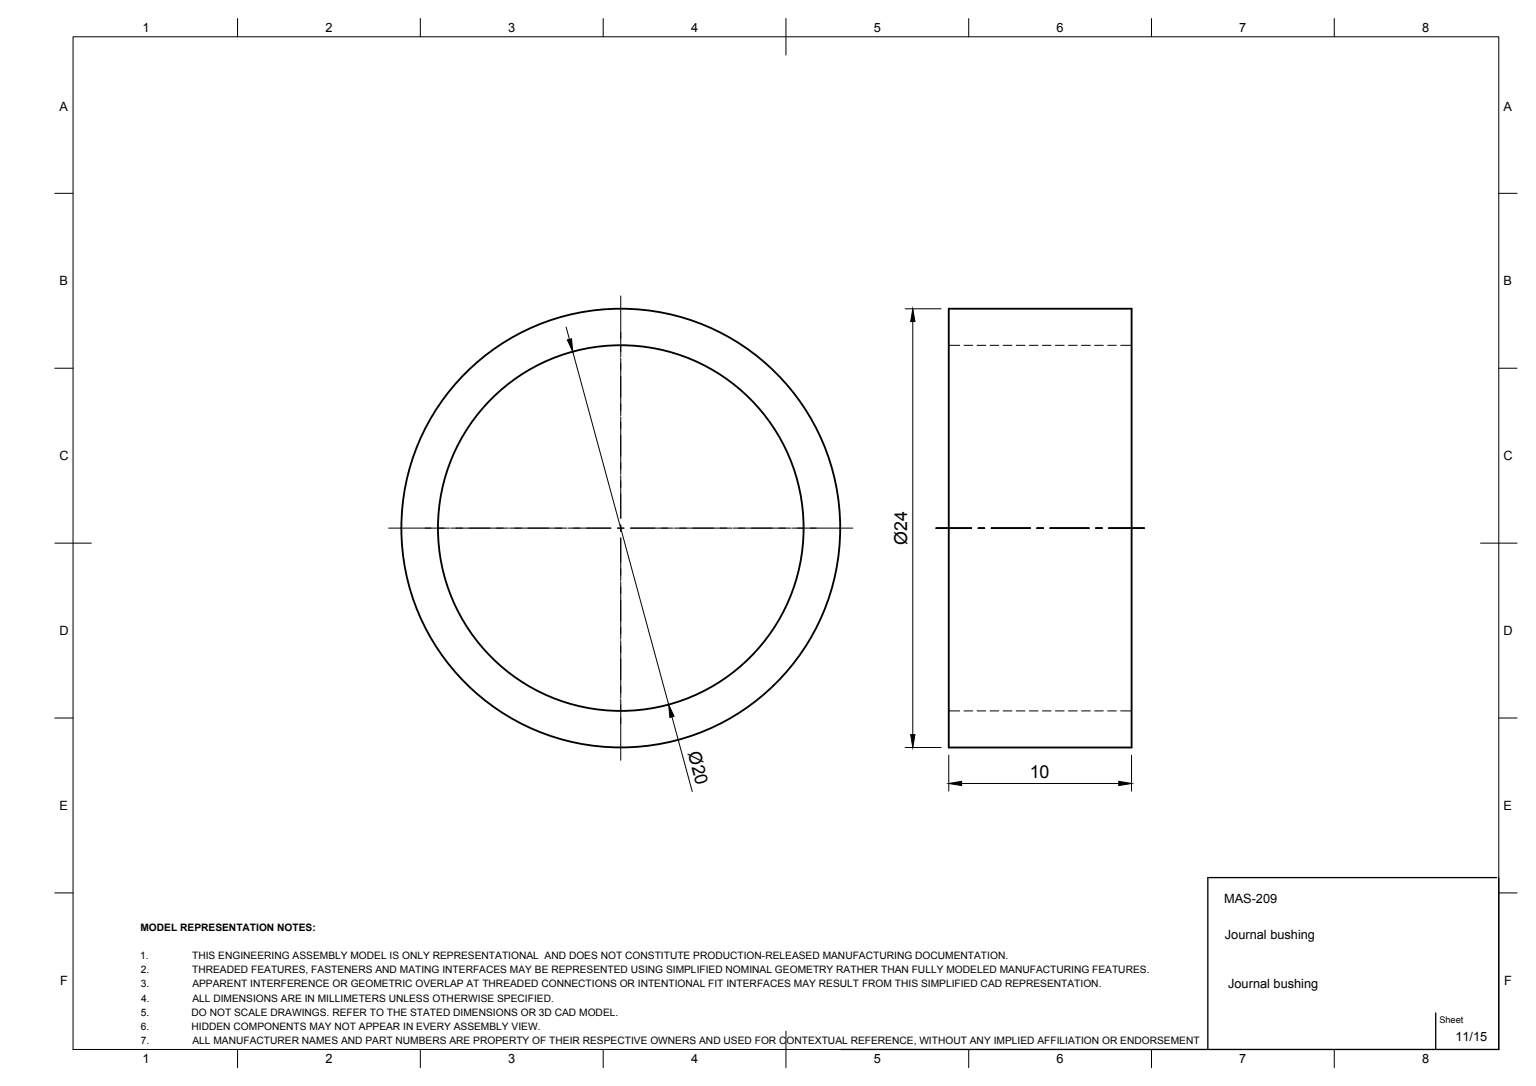
ISO-10303-21;
HEADER;
/* Generated by software containing ST-Developer
 * from STEP Tools, Inc. (www.steptools.com) 
 */

FILE_DESCRIPTION(
/* description */ ('Independent bearing-supported roller-ramp one-way clutch. Six logarit
hmic ramps with plain solid rollers, sprung guided plungers, native Co
il variants, removable shared keepers, rounded parallel key, shaft wit
h complete retaining lips, bronze journal/thrust support and bolted co
vers. Native rotor, roller planar/spin and plunger joints permit manua
l geometric engaged/released inspection. Automatic frictional torque s
witching/contact dynamics are not simulated; no capacity, hardness, fi
t, lubrication, speed, force or life rating. External input driver/cou
pling/anchors outside assembly.'),
/* implementation_level */ '2;1');

FILE_NAME(
/* name */ 'Journal bushing.step',
/* time_stamp */ '2026-11-08T07:04:38-08:00',
/* author */ (''),
/* organization */ (''),
/* preprocessor_version */ 'ST-DEVELOPER v20.2',
/* originating_system */ 'Autodesk Translation Framework v15.17.0.0',
/* authorisation */ '');

FILE_SCHEMA (('AUTOMOTIVE_DESIGN { 1 0 10303 214 3 1 1 }'));
ENDSEC;

DATA;
#10=MECHANICAL_DESIGN_GEOMETRIC_PRESENTATION_REPRESENTATION('',(#308),#99526);
#276=SHAPE_REPRESENTATION_RELATIONSHIP('SRR','None',#99633,#292);
#292=ADVANCED_BREP_SHAPE_REPRESENTATION('',(#324),#99518);
#308=STYLED_ITEM('',(#99720),#324);
#324=MANIFOLD_SOLID_BREP('Body1',#18278);
#430=FACE_BOUND('',#2664,.T.);
#431=FACE_BOUND('',#2666,.T.);
#579=PLANE('',#19601);
#580=PLANE('',#19602);
#1566=FACE_OUTER_BOUND('',#2661,.T.);
#1567=FACE_OUTER_BOUND('',#2662,.T.);
#1568=FACE_OUTER_BOUND('',#2663,.T.);
#1569=FACE_OUTER_BOUND('',#2665,.T.);
#2661=EDGE_LOOP('',(#16020,#16021,#16022,#16023));
#2662=EDGE_LOOP('',(#16024,#16025,#16026,#16027));
#2663=EDGE_LOOP('',(#16028));
#2664=EDGE_LOOP('',(#16029));
#2665=EDGE_LOOP('',(#16030));
#2666=EDGE_LOOP('',(#16031));
#3076=CIRCLE('',#19596,10.);
#3077=CIRCLE('',#19597,10.);
#3078=CIRCLE('',#19599,12.);
#3079=CIRCLE('',#19600,12.);
#5430=LINE('',#94854,#6334);
#5431=LINE('',#94860,#6335);
#6334=VECTOR('',#22867,10.);
#6335=VECTOR('',#22874,12.);
#8091=VERTEX_POINT('',#94851);
#8092=VERTEX_POINT('',#94853);
#8093=VERTEX_POINT('',#94857);
#8094=VERTEX_POINT('',#94859);
#10762=EDGE_CURVE('',#8091,#8091,#3076,.T.);
#10763=EDGE_CURVE('',#8091,#8092,#5430,.T.);
#10764=EDGE_CURVE('',#8092,#8092,#3077,.T.);
#10765=EDGE_CURVE('',#8093,#8093,#3078,.T.);
#10766=EDGE_CURVE('',#8093,#8094,#5431,.T.);
#10767=EDGE_CURVE('',#8094,#8094,#3079,.T.);
#16020=ORIENTED_EDGE('',*,*,#10762,.F.);
#16021=ORIENTED_EDGE('',*,*,#10763,.T.);
#16022=ORIENTED_EDGE('',*,*,#10764,.T.);
#16023=ORIENTED_EDGE('',*,*,#10763,.F.);
#16024=ORIENTED_EDGE('',*,*,#10765,.F.);
#16025=ORIENTED_EDGE('',*,*,#10766,.T.);
#16026=ORIENTED_EDGE('',*,*,#10767,.T.);
#16027=ORIENTED_EDGE('',*,*,#10766,.F.);
#16028=ORIENTED_EDGE('',*,*,#10765,.T.);
#16029=ORIENTED_EDGE('',*,*,#10762,.T.);
#16030=ORIENTED_EDGE('',*,*,#10767,.F.);
#16031=ORIENTED_EDGE('',*,*,#10764,.F.);
#17210=CYLINDRICAL_SURFACE('',#19595,10.);
#17211=CYLINDRICAL_SURFACE('',#19598,12.);
#18164=ADVANCED_FACE('',(#1566),#17210,.F.);
#18165=ADVANCED_FACE('',(#1567),#17211,.T.);
#18166=ADVANCED_FACE('',(#1568,#430),#579,.T.);
#18167=ADVANCED_FACE('',(#1569,#431),#580,.F.);
#18278=CLOSED_SHELL('',(#18164,#18165,#18166,#18167));
#19594=AXIS2_PLACEMENT_3D('',#94849,#22861,#22862);
#19595=AXIS2_PLACEMENT_3D('',#94850,#22863,#22864);
#19596=AXIS2_PLACEMENT_3D('',#94852,#22865,#22866);
#19597=AXIS2_PLACEMENT_3D('',#94855,#22868,#22869);
#19598=AXIS2_PLACEMENT_3D('',#94856,#22870,#22871);
#19599=AXIS2_PLACEMENT_3D('',#94858,#22872,#22873);
#19600=AXIS2_PLACEMENT_3D('',#94861,#22875,#22876);
#19601=AXIS2_PLACEMENT_3D('',#94862,#22877,#22878);
#19602=AXIS2_PLACEMENT_3D('',#94863,#22879,#22880);
#22861=DIRECTION('axis',(0.,0.,1.));
#22862=DIRECTION('refdir',(1.,0.,0.));
#22863=DIRECTION('center_axis',(0.,0.,1.));
#22864=DIRECTION('ref_axis',(1.,0.,0.));
#22865=DIRECTION('center_axis',(0.,0.,-1.));
#22866=DIRECTION('ref_axis',(1.,0.,0.));
#22867=DIRECTION('',(0.,0.,-1.));
#22868=DIRECTION('center_axis',(0.,0.,-1.));
#22869=DIRECTION('ref_axis',(1.,0.,0.));
#22870=DIRECTION('center_axis',(0.,0.,1.));
#22871=DIRECTION('ref_axis',(1.,0.,0.));
#22872=DIRECTION('center_axis',(0.,0.,1.));
#22873=DIRECTION('ref_axis',(1.,0.,0.));
#22874=DIRECTION('',(0.,0.,-1.));
#22875=DIRECTION('center_axis',(0.,0.,1.));
#22876=DIRECTION('ref_axis',(1.,0.,0.));
#22877=DIRECTION('center_axis',(0.,0.,1.));
#22878=DIRECTION('ref_axis',(1.,0.,0.));
#22879=DIRECTION('center_axis',(0.,0.,1.));
#22880=DIRECTION('ref_axis',(1.,0.,0.));
#94849=CARTESIAN_POINT('',(0.,0.,0.));
#94850=CARTESIAN_POINT('Origin',(0.,0.,0.));
#94851=CARTESIAN_POINT('',(-10.,-1.22464679914735E-15,10.));
#94852=CARTESIAN_POINT('Origin',(0.,0.,10.));
#94853=CARTESIAN_POINT('',(-10.,-1.22464679914735E-15,0.));
#94854=CARTESIAN_POINT('',(-10.,-1.22464679914735E-15,0.));
#94855=CARTESIAN_POINT('Origin',(0.,0.,0.));
#94856=CARTESIAN_POINT('Origin',(0.,0.,0.));
#94857=CARTESIAN_POINT('',(-12.,-1.46957615897682E-15,10.));
#94858=CARTESIAN_POINT('Origin',(0.,0.,10.));
#94859=CARTESIAN_POINT('',(-12.,-1.46957615897682E-15,0.));
#94860=CARTESIAN_POINT('',(-12.,-1.46957615897682E-15,0.));
#94861=CARTESIAN_POINT('Origin',(0.,0.,0.));
#94862=CARTESIAN_POINT('Origin',(0.,0.,10.));
#94863=CARTESIAN_POINT('Origin',(0.,0.,0.));
#99500=UNCERTAINTY_MEASURE_WITH_UNIT(LENGTH_MEASURE(0.01),#99527,
'DISTANCE_ACCURACY_VALUE',
'Maximum model space distance between geometric entities at asserted c
onnectivities');
#99508=UNCERTAINTY_MEASURE_WITH_UNIT(LENGTH_MEASURE(0.01),#99527,
'DISTANCE_ACCURACY_VALUE',
'Maximum model space distance between geometric entities at asserted c
onnectivities');
#99518=(
GEOMETRIC_REPRESENTATION_CONTEXT(3)
GLOBAL_UNCERTAINTY_ASSIGNED_CONTEXT((#99500))
GLOBAL_UNIT_ASSIGNED_CONTEXT((#99527,#99529,#99530))
REPRESENTATION_CONTEXT('','3D')
);
#99526=(
GEOMETRIC_REPRESENTATION_CONTEXT(3)
GLOBAL_UNCERTAINTY_ASSIGNED_CONTEXT((#99508))
GLOBAL_UNIT_ASSIGNED_CONTEXT((#99527,#99529,#99530))
REPRESENTATION_CONTEXT('','3D')
);
#99527=(
LENGTH_UNIT()
NAMED_UNIT(*)
SI_UNIT(.MILLI.,.METRE.)
);
#99529=(
NAMED_UNIT(*)
PLANE_ANGLE_UNIT()
SI_UNIT($,.RADIAN.)
);
#99530=(
NAMED_UNIT(*)
SI_UNIT($,.STERADIAN.)
SOLID_ANGLE_UNIT()
);
#99540=SHAPE_DEFINITION_REPRESENTATION(#99557,#99633);
#99557=PRODUCT_DEFINITION_SHAPE('',$,#99651);
#99633=SHAPE_REPRESENTATION('',(#19594),#99518);
#99641=PRODUCT_DEFINITION_CONTEXT('part definition',#99694,'design');
#99651=PRODUCT_DEFINITION('Journal bushing','Journal bushing',#99668,#99641);
#99668=PRODUCT_DEFINITION_FORMATION('',$,#99705);
#99694=APPLICATION_CONTEXT(
'Core Data for Automotive Mechanical Design Process');
#99695=PRODUCT_CONTEXT('part definition',#99694,'mechanical');
#99705=PRODUCT('Journal bushing','Journal bushing',$,(#99695));
#99720=PRESENTATION_STYLE_ASSIGNMENT((#99733));
#99733=SURFACE_STYLE_USAGE(.BOTH.,#99746);
#99746=SURFACE_SIDE_STYLE('',(#99759));
#99759=SURFACE_STYLE_FILL_AREA(#99772);
#99772=FILL_AREA_STYLE('Bearing light gray',(#99785));
#99785=FILL_AREA_STYLE_COLOUR('Bearing light gray',#99798);
#99798=COLOUR_RGB('Bearing light gray',0.725490196078431,0.752941176470588,
0.792156862745098);
ENDSEC;
END-ISO-10303-21;
